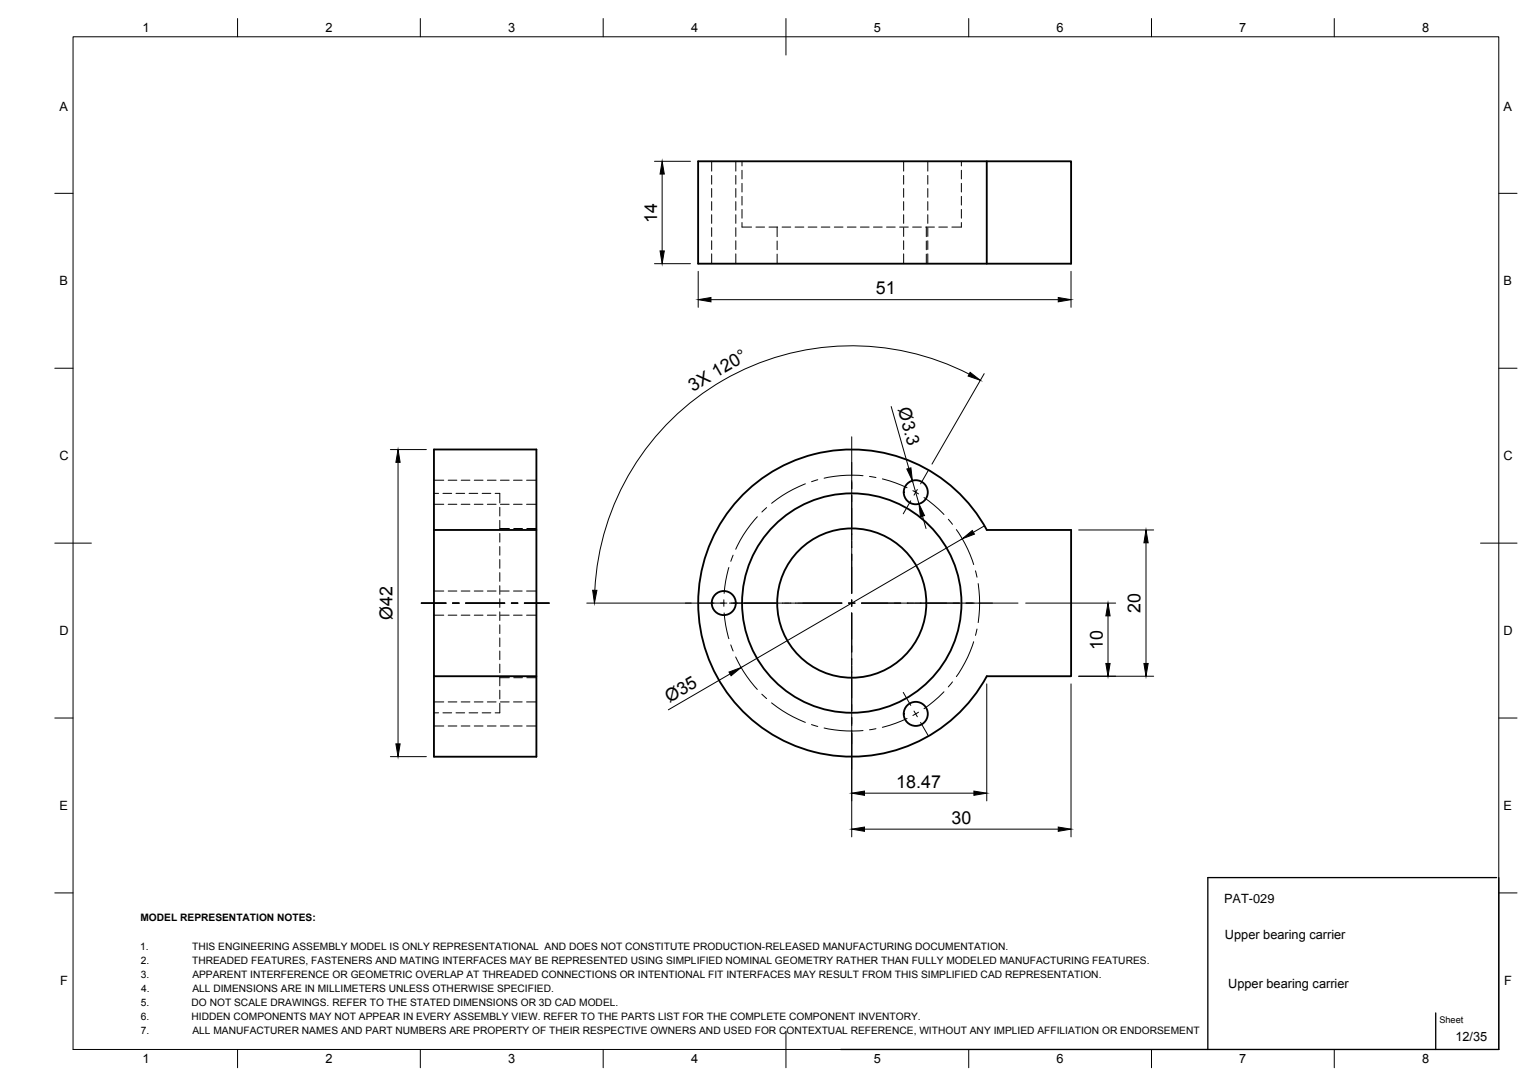
ISO-10303-21;
HEADER;
/* Generated by software containing ST-Developer
 * from STEP Tools, Inc. (www.steptools.com) 
 */

FILE_DESCRIPTION(
/* description */ ('Door-style hinge test fixture with detent'),
/* implementation_level */ '2;1');

FILE_NAME(
/* name */ 'Upper bearing carrier.step',
/* time_stamp */ '2026-10-28T03:24:57-07:00',
/* author */ (''),
/* organization */ (''),
/* preprocessor_version */ 'ST-DEVELOPER v20.2',
/* originating_system */ 'Autodesk Translation Framework v15.17.0.0',
/* authorisation */ '');

FILE_SCHEMA (('AUTOMOTIVE_DESIGN { 1 0 10303 214 3 1 1 }'));
ENDSEC;

DATA;
#10=MECHANICAL_DESIGN_GEOMETRIC_PRESENTATION_REPRESENTATION('',(#330),#9813);
#267=SHAPE_REPRESENTATION_RELATIONSHIP('SRR','None',#9944,#298);
#298=ADVANCED_BREP_SHAPE_REPRESENTATION('',(#370),#9787);
#330=STYLED_ITEM('',(#10183),#370);
#370=MANIFOLD_SOLID_BREP('Body1',#4761);
#440=FACE_BOUND('',#1067,.T.);
#441=FACE_BOUND('',#1070,.T.);
#442=FACE_BOUND('',#1071,.T.);
#443=FACE_BOUND('',#1072,.T.);
#444=FACE_BOUND('',#1073,.T.);
#445=FACE_BOUND('',#1079,.T.);
#446=FACE_BOUND('',#1080,.T.);
#447=FACE_BOUND('',#1081,.T.);
#448=FACE_BOUND('',#1082,.T.);
#547=PLANE('',#5291);
#548=PLANE('',#5295);
#549=PLANE('',#5297);
#550=PLANE('',#5298);
#551=PLANE('',#5299);
#552=PLANE('',#5302);
#736=FACE_OUTER_BOUND('',#1062,.T.);
#737=FACE_OUTER_BOUND('',#1063,.T.);
#738=FACE_OUTER_BOUND('',#1064,.T.);
#739=FACE_OUTER_BOUND('',#1065,.T.);
#740=FACE_OUTER_BOUND('',#1066,.T.);
#741=FACE_OUTER_BOUND('',#1068,.T.);
#742=FACE_OUTER_BOUND('',#1069,.T.);
#743=FACE_OUTER_BOUND('',#1074,.T.);
#744=FACE_OUTER_BOUND('',#1075,.T.);
#745=FACE_OUTER_BOUND('',#1076,.T.);
#746=FACE_OUTER_BOUND('',#1077,.T.);
#747=FACE_OUTER_BOUND('',#1078,.T.);
#1062=EDGE_LOOP('',(#3543,#3544,#3545,#3546));
#1063=EDGE_LOOP('',(#3547,#3548,#3549,#3550));
#1064=EDGE_LOOP('',(#3551,#3552,#3553,#3554));
#1065=EDGE_LOOP('',(#3555,#3556,#3557,#3558));
#1066=EDGE_LOOP('',(#3559));
#1067=EDGE_LOOP('',(#3560));
#1068=EDGE_LOOP('',(#3561,#3562,#3563,#3564));
#1069=EDGE_LOOP('',(#3565,#3566,#3567,#3568));
#1070=EDGE_LOOP('',(#3569));
#1071=EDGE_LOOP('',(#3570));
#1072=EDGE_LOOP('',(#3571));
#1073=EDGE_LOOP('',(#3572));
#1074=EDGE_LOOP('',(#3573,#3574,#3575,#3576));
#1075=EDGE_LOOP('',(#3577,#3578,#3579,#3580));
#1076=EDGE_LOOP('',(#3581,#3582,#3583,#3584));
#1077=EDGE_LOOP('',(#3585,#3586,#3587,#3588));
#1078=EDGE_LOOP('',(#3589,#3590,#3591,#3592));
#1079=EDGE_LOOP('',(#3593));
#1080=EDGE_LOOP('',(#3594));
#1081=EDGE_LOOP('',(#3595));
#1082=EDGE_LOOP('',(#3596));
#1444=LINE('',#7664,#1764);
#1445=LINE('',#7670,#1765);
#1446=LINE('',#7676,#1766);
#1447=LINE('',#7682,#1767);
#1448=LINE('',#7689,#1768);
#1449=LINE('',#7694,#1769);
#1450=LINE('',#7696,#1770);
#1451=LINE('',#7698,#1771);
#1452=LINE('',#7702,#1772);
#1453=LINE('',#7704,#1773);
#1454=LINE('',#7705,#1774);
#1455=LINE('',#7708,#1775);
#1456=LINE('',#7710,#1776);
#1457=LINE('',#7711,#1777);
#1458=LINE('',#7713,#1778);
#1764=VECTOR('',#6147,0.165);
#1765=VECTOR('',#6154,0.165);
#1766=VECTOR('',#6161,0.165);
#1767=VECTOR('',#6168,1.5);
#1768=VECTOR('',#6177,1.02);
#1769=VECTOR('',#6182,1.);
#1770=VECTOR('',#6183,1.);
#1771=VECTOR('',#6184,1.);
#1772=VECTOR('',#6189,1.);
#1773=VECTOR('',#6190,1.);
#1774=VECTOR('',#6191,1.);
#1775=VECTOR('',#6194,1.);
#1776=VECTOR('',#6195,1.);
#1777=VECTOR('',#6196,1.);
#1778=VECTOR('',#6199,1.);
#2032=CIRCLE('',#5280,0.165);
#2033=CIRCLE('',#5281,0.165);
#2034=CIRCLE('',#5283,0.165);
#2035=CIRCLE('',#5284,0.165);
#2036=CIRCLE('',#5286,0.165);
#2037=CIRCLE('',#5287,0.165);
#2038=CIRCLE('',#5289,1.5);
#2039=CIRCLE('',#5290,1.5);
#2040=CIRCLE('',#5292,1.02);
#2041=CIRCLE('',#5294,1.02);
#2042=CIRCLE('',#5296,2.1);
#2043=CIRCLE('',#5301,2.1);
#2333=VERTEX_POINT('',#7661);
#2334=VERTEX_POINT('',#7663);
#2335=VERTEX_POINT('',#7667);
#2336=VERTEX_POINT('',#7669);
#2337=VERTEX_POINT('',#7673);
#2338=VERTEX_POINT('',#7675);
#2339=VERTEX_POINT('',#7679);
#2340=VERTEX_POINT('',#7681);
#2341=VERTEX_POINT('',#7685);
#2342=VERTEX_POINT('',#7688);
#2343=VERTEX_POINT('',#7692);
#2344=VERTEX_POINT('',#7693);
#2345=VERTEX_POINT('',#7695);
#2346=VERTEX_POINT('',#7697);
#2347=VERTEX_POINT('',#7701);
#2348=VERTEX_POINT('',#7703);
#2349=VERTEX_POINT('',#7707);
#2350=VERTEX_POINT('',#7709);
#2788=EDGE_CURVE('',#2333,#2333,#2032,.T.);
#2789=EDGE_CURVE('',#2333,#2334,#1444,.T.);
#2790=EDGE_CURVE('',#2334,#2334,#2033,.T.);
#2791=EDGE_CURVE('',#2335,#2335,#2034,.T.);
#2792=EDGE_CURVE('',#2335,#2336,#1445,.T.);
#2793=EDGE_CURVE('',#2336,#2336,#2035,.T.);
#2794=EDGE_CURVE('',#2337,#2337,#2036,.T.);
#2795=EDGE_CURVE('',#2337,#2338,#1446,.T.);
#2796=EDGE_CURVE('',#2338,#2338,#2037,.T.);
#2797=EDGE_CURVE('',#2339,#2339,#2038,.T.);
#2798=EDGE_CURVE('',#2339,#2340,#1447,.T.);
#2799=EDGE_CURVE('',#2340,#2340,#2039,.T.);
#2800=EDGE_CURVE('',#2341,#2341,#2040,.T.);
#2801=EDGE_CURVE('',#2341,#2342,#1448,.T.);
#2802=EDGE_CURVE('',#2342,#2342,#2041,.T.);
#2803=EDGE_CURVE('',#2343,#2344,#1449,.T.);
#2804=EDGE_CURVE('',#2344,#2345,#1450,.T.);
#2805=EDGE_CURVE('',#2345,#2346,#1451,.T.);
#2806=EDGE_CURVE('',#2346,#2343,#2042,.T.);
#2807=EDGE_CURVE('',#2347,#2343,#1452,.T.);
#2808=EDGE_CURVE('',#2347,#2348,#1453,.T.);
#2809=EDGE_CURVE('',#2348,#2344,#1454,.T.);
#2810=EDGE_CURVE('',#2346,#2349,#1455,.T.);
#2811=EDGE_CURVE('',#2350,#2345,#1456,.T.);
#2812=EDGE_CURVE('',#2350,#2349,#1457,.T.);
#2813=EDGE_CURVE('',#2348,#2350,#1458,.T.);
#2814=EDGE_CURVE('',#2349,#2347,#2043,.T.);
#3543=ORIENTED_EDGE('',*,*,#2788,.F.);
#3544=ORIENTED_EDGE('',*,*,#2789,.T.);
#3545=ORIENTED_EDGE('',*,*,#2790,.F.);
#3546=ORIENTED_EDGE('',*,*,#2789,.F.);
#3547=ORIENTED_EDGE('',*,*,#2791,.F.);
#3548=ORIENTED_EDGE('',*,*,#2792,.T.);
#3549=ORIENTED_EDGE('',*,*,#2793,.F.);
#3550=ORIENTED_EDGE('',*,*,#2792,.F.);
#3551=ORIENTED_EDGE('',*,*,#2794,.F.);
#3552=ORIENTED_EDGE('',*,*,#2795,.T.);
#3553=ORIENTED_EDGE('',*,*,#2796,.F.);
#3554=ORIENTED_EDGE('',*,*,#2795,.F.);
#3555=ORIENTED_EDGE('',*,*,#2797,.F.);
#3556=ORIENTED_EDGE('',*,*,#2798,.T.);
#3557=ORIENTED_EDGE('',*,*,#2799,.T.);
#3558=ORIENTED_EDGE('',*,*,#2798,.F.);
#3559=ORIENTED_EDGE('',*,*,#2799,.F.);
#3560=ORIENTED_EDGE('',*,*,#2800,.F.);
#3561=ORIENTED_EDGE('',*,*,#2800,.T.);
#3562=ORIENTED_EDGE('',*,*,#2801,.T.);
#3563=ORIENTED_EDGE('',*,*,#2802,.F.);
#3564=ORIENTED_EDGE('',*,*,#2801,.F.);
#3565=ORIENTED_EDGE('',*,*,#2803,.T.);
#3566=ORIENTED_EDGE('',*,*,#2804,.T.);
#3567=ORIENTED_EDGE('',*,*,#2805,.T.);
#3568=ORIENTED_EDGE('',*,*,#2806,.T.);
#3569=ORIENTED_EDGE('',*,*,#2790,.T.);
#3570=ORIENTED_EDGE('',*,*,#2793,.T.);
#3571=ORIENTED_EDGE('',*,*,#2796,.T.);
#3572=ORIENTED_EDGE('',*,*,#2802,.T.);
#3573=ORIENTED_EDGE('',*,*,#2807,.F.);
#3574=ORIENTED_EDGE('',*,*,#2808,.T.);
#3575=ORIENTED_EDGE('',*,*,#2809,.T.);
#3576=ORIENTED_EDGE('',*,*,#2803,.F.);
#3577=ORIENTED_EDGE('',*,*,#2810,.F.);
#3578=ORIENTED_EDGE('',*,*,#2805,.F.);
#3579=ORIENTED_EDGE('',*,*,#2811,.F.);
#3580=ORIENTED_EDGE('',*,*,#2812,.T.);
#3581=ORIENTED_EDGE('',*,*,#2813,.T.);
#3582=ORIENTED_EDGE('',*,*,#2811,.T.);
#3583=ORIENTED_EDGE('',*,*,#2804,.F.);
#3584=ORIENTED_EDGE('',*,*,#2809,.F.);
#3585=ORIENTED_EDGE('',*,*,#2807,.T.);
#3586=ORIENTED_EDGE('',*,*,#2806,.F.);
#3587=ORIENTED_EDGE('',*,*,#2810,.T.);
#3588=ORIENTED_EDGE('',*,*,#2814,.T.);
#3589=ORIENTED_EDGE('',*,*,#2814,.F.);
#3590=ORIENTED_EDGE('',*,*,#2812,.F.);
#3591=ORIENTED_EDGE('',*,*,#2813,.F.);
#3592=ORIENTED_EDGE('',*,*,#2808,.F.);
#3593=ORIENTED_EDGE('',*,*,#2788,.T.);
#3594=ORIENTED_EDGE('',*,*,#2791,.T.);
#3595=ORIENTED_EDGE('',*,*,#2794,.T.);
#3596=ORIENTED_EDGE('',*,*,#2797,.T.);
#4407=CYLINDRICAL_SURFACE('',#5279,0.165);
#4408=CYLINDRICAL_SURFACE('',#5282,0.165);
#4409=CYLINDRICAL_SURFACE('',#5285,0.165);
#4410=CYLINDRICAL_SURFACE('',#5288,1.5);
#4411=CYLINDRICAL_SURFACE('',#5293,1.02);
#4412=CYLINDRICAL_SURFACE('',#5300,2.1);
#4541=ADVANCED_FACE('',(#736),#4407,.F.);
#4542=ADVANCED_FACE('',(#737),#4408,.F.);
#4543=ADVANCED_FACE('',(#738),#4409,.F.);
#4544=ADVANCED_FACE('',(#739),#4410,.F.);
#4545=ADVANCED_FACE('',(#740,#440),#547,.F.);
#4546=ADVANCED_FACE('',(#741),#4411,.F.);
#4547=ADVANCED_FACE('',(#742,#441,#442,#443,#444),#548,.T.);
#4548=ADVANCED_FACE('',(#743),#549,.T.);
#4549=ADVANCED_FACE('',(#744),#550,.T.);
#4550=ADVANCED_FACE('',(#745),#551,.T.);
#4551=ADVANCED_FACE('',(#746),#4412,.T.);
#4552=ADVANCED_FACE('',(#747,#445,#446,#447,#448),#552,.F.);
#4761=CLOSED_SHELL('',(#4541,#4542,#4543,#4544,#4545,#4546,#4547,#4548,
#4549,#4550,#4551,#4552));
#5278=AXIS2_PLACEMENT_3D('',#7659,#6141,#6142);
#5279=AXIS2_PLACEMENT_3D('',#7660,#6143,#6144);
#5280=AXIS2_PLACEMENT_3D('',#7662,#6145,#6146);
#5281=AXIS2_PLACEMENT_3D('',#7665,#6148,#6149);
#5282=AXIS2_PLACEMENT_3D('',#7666,#6150,#6151);
#5283=AXIS2_PLACEMENT_3D('',#7668,#6152,#6153);
#5284=AXIS2_PLACEMENT_3D('',#7671,#6155,#6156);
#5285=AXIS2_PLACEMENT_3D('',#7672,#6157,#6158);
#5286=AXIS2_PLACEMENT_3D('',#7674,#6159,#6160);
#5287=AXIS2_PLACEMENT_3D('',#7677,#6162,#6163);
#5288=AXIS2_PLACEMENT_3D('',#7678,#6164,#6165);
#5289=AXIS2_PLACEMENT_3D('',#7680,#6166,#6167);
#5290=AXIS2_PLACEMENT_3D('',#7683,#6169,#6170);
#5291=AXIS2_PLACEMENT_3D('',#7684,#6171,#6172);
#5292=AXIS2_PLACEMENT_3D('',#7686,#6173,#6174);
#5293=AXIS2_PLACEMENT_3D('',#7687,#6175,#6176);
#5294=AXIS2_PLACEMENT_3D('',#7690,#6178,#6179);
#5295=AXIS2_PLACEMENT_3D('',#7691,#6180,#6181);
#5296=AXIS2_PLACEMENT_3D('',#7699,#6185,#6186);
#5297=AXIS2_PLACEMENT_3D('',#7700,#6187,#6188);
#5298=AXIS2_PLACEMENT_3D('',#7706,#6192,#6193);
#5299=AXIS2_PLACEMENT_3D('',#7712,#6197,#6198);
#5300=AXIS2_PLACEMENT_3D('',#7714,#6200,#6201);
#5301=AXIS2_PLACEMENT_3D('',#7715,#6202,#6203);
#5302=AXIS2_PLACEMENT_3D('',#7716,#6204,#6205);
#6141=DIRECTION('axis',(0.,0.,1.));
#6142=DIRECTION('refdir',(1.,0.,0.));
#6143=DIRECTION('center_axis',(0.,0.,1.));
#6144=DIRECTION('ref_axis',(1.,0.,0.));
#6145=DIRECTION('center_axis',(0.,0.,1.));
#6146=DIRECTION('ref_axis',(1.,0.,0.));
#6147=DIRECTION('',(0.,0.,1.));
#6148=DIRECTION('center_axis',(0.,0.,-1.));
#6149=DIRECTION('ref_axis',(1.,0.,0.));
#6150=DIRECTION('center_axis',(0.,0.,1.));
#6151=DIRECTION('ref_axis',(1.,0.,0.));
#6152=DIRECTION('center_axis',(0.,0.,1.));
#6153=DIRECTION('ref_axis',(1.,0.,0.));
#6154=DIRECTION('',(0.,0.,1.));
#6155=DIRECTION('center_axis',(0.,0.,-1.));
#6156=DIRECTION('ref_axis',(1.,0.,0.));
#6157=DIRECTION('center_axis',(0.,0.,1.));
#6158=DIRECTION('ref_axis',(1.,0.,0.));
#6159=DIRECTION('center_axis',(0.,0.,1.));
#6160=DIRECTION('ref_axis',(1.,0.,0.));
#6161=DIRECTION('',(0.,0.,1.));
#6162=DIRECTION('center_axis',(0.,0.,-1.));
#6163=DIRECTION('ref_axis',(1.,0.,0.));
#6164=DIRECTION('center_axis',(0.,0.,1.));
#6165=DIRECTION('ref_axis',(1.,0.,0.));
#6166=DIRECTION('center_axis',(0.,0.,1.));
#6167=DIRECTION('ref_axis',(1.,0.,0.));
#6168=DIRECTION('',(0.,0.,1.));
#6169=DIRECTION('center_axis',(0.,0.,1.));
#6170=DIRECTION('ref_axis',(1.,0.,0.));
#6171=DIRECTION('center_axis',(0.,0.,1.));
#6172=DIRECTION('ref_axis',(1.,0.,0.));
#6173=DIRECTION('center_axis',(0.,0.,-1.));
#6174=DIRECTION('ref_axis',(1.,0.,0.));
#6175=DIRECTION('center_axis',(0.,0.,1.));
#6176=DIRECTION('ref_axis',(1.,0.,0.));
#6177=DIRECTION('',(0.,0.,1.));
#6178=DIRECTION('center_axis',(0.,0.,-1.));
#6179=DIRECTION('ref_axis',(1.,0.,0.));
#6180=DIRECTION('center_axis',(0.,0.,1.));
#6181=DIRECTION('ref_axis',(1.,0.,0.));
#6182=DIRECTION('',(-1.,0.,0.));
#6183=DIRECTION('',(0.,-1.,0.));
#6184=DIRECTION('',(1.,0.,0.));
#6185=DIRECTION('center_axis',(0.,0.,1.));
#6186=DIRECTION('ref_axis',(1.,0.,0.));
#6187=DIRECTION('center_axis',(0.,1.,0.));
#6188=DIRECTION('ref_axis',(-1.,0.,0.));
#6189=DIRECTION('',(0.,0.,1.));
#6190=DIRECTION('',(-1.,0.,0.));
#6191=DIRECTION('',(0.,0.,1.));
#6192=DIRECTION('center_axis',(0.,-1.,0.));
#6193=DIRECTION('ref_axis',(1.,0.,0.));
#6194=DIRECTION('',(0.,0.,-1.));
#6195=DIRECTION('',(0.,0.,1.));
#6196=DIRECTION('',(1.,0.,0.));
#6197=DIRECTION('center_axis',(-1.,0.,0.));
#6198=DIRECTION('ref_axis',(0.,-1.,0.));
#6199=DIRECTION('',(0.,-1.,0.));
#6200=DIRECTION('center_axis',(0.,0.,1.));
#6201=DIRECTION('ref_axis',(1.,0.,0.));
#6202=DIRECTION('center_axis',(0.,0.,1.));
#6203=DIRECTION('ref_axis',(1.,0.,0.));
#6204=DIRECTION('center_axis',(0.,0.,1.));
#6205=DIRECTION('ref_axis',(1.,0.,0.));
#7659=CARTESIAN_POINT('',(0.,0.,0.));
#7660=CARTESIAN_POINT('Origin',(1.75,0.,10.5));
#7661=CARTESIAN_POINT('',(1.585,-2.02066721859313E-17,10.6));
#7662=CARTESIAN_POINT('Origin',(1.75,0.,10.6));
#7663=CARTESIAN_POINT('',(1.585,2.02066721859313E-17,12.));
#7664=CARTESIAN_POINT('',(1.585,-2.02066721859313E-17,10.5));
#7665=CARTESIAN_POINT('Origin',(1.75,0.,12.));
#7666=CARTESIAN_POINT('Origin',(-0.875,1.51554445662277,10.5));
#7667=CARTESIAN_POINT('',(-1.04,1.51554445662277,10.6));
#7668=CARTESIAN_POINT('Origin',(-0.875,1.51554445662277,10.6));
#7669=CARTESIAN_POINT('',(-1.04,1.51554445662277,12.));
#7670=CARTESIAN_POINT('',(-1.04,1.51554445662277,10.5));
#7671=CARTESIAN_POINT('Origin',(-0.875,1.51554445662277,12.));
#7672=CARTESIAN_POINT('Origin',(-0.875000000000001,-1.51554445662277,10.5));
#7673=CARTESIAN_POINT('',(-1.04,-1.51554445662277,10.6));
#7674=CARTESIAN_POINT('Origin',(-0.875000000000001,-1.51554445662277,10.6));
#7675=CARTESIAN_POINT('',(-1.04,-1.51554445662277,12.));
#7676=CARTESIAN_POINT('',(-1.04,-1.51554445662277,10.5));
#7677=CARTESIAN_POINT('Origin',(-0.875000000000001,-1.51554445662277,12.));
#7678=CARTESIAN_POINT('Origin',(0.,0.,10.5));
#7679=CARTESIAN_POINT('',(-1.5,-1.83697019872103E-16,10.6));
#7680=CARTESIAN_POINT('Origin',(0.,0.,10.6));
#7681=CARTESIAN_POINT('',(-1.5,-1.83697019872103E-16,11.5));
#7682=CARTESIAN_POINT('',(-1.5,-1.83697019872103E-16,10.5));
#7683=CARTESIAN_POINT('Origin',(0.,0.,11.5));
#7684=CARTESIAN_POINT('Origin',(0.,0.,11.5));
#7685=CARTESIAN_POINT('',(-1.02,1.2491397351303E-16,11.5));
#7686=CARTESIAN_POINT('Origin',(0.,0.,11.5));
#7687=CARTESIAN_POINT('Origin',(0.,0.,10.5));
#7688=CARTESIAN_POINT('',(-1.02,1.2491397351303E-16,12.));
#7689=CARTESIAN_POINT('',(-1.02,-1.2491397351303E-16,10.5));
#7690=CARTESIAN_POINT('Origin',(0.,0.,12.));
#7691=CARTESIAN_POINT('Origin',(0.,0.,12.));
#7692=CARTESIAN_POINT('',(-1.84661853126194,1.,12.));
#7693=CARTESIAN_POINT('',(-3.,1.,12.));
#7694=CARTESIAN_POINT('',(0.,1.,12.));
#7695=CARTESIAN_POINT('',(-3.,-1.,12.));
#7696=CARTESIAN_POINT('',(-3.,1.,12.));
#7697=CARTESIAN_POINT('',(-1.84661853126194,-1.,12.));
#7698=CARTESIAN_POINT('',(-3.,-1.,12.));
#7699=CARTESIAN_POINT('Origin',(0.,0.,12.));
#7700=CARTESIAN_POINT('Origin',(0.,1.,10.6));
#7701=CARTESIAN_POINT('',(-1.84661853126194,1.,10.6));
#7702=CARTESIAN_POINT('',(-1.84661853126194,1.,10.6));
#7703=CARTESIAN_POINT('',(-3.,1.,10.6));
#7704=CARTESIAN_POINT('',(0.,1.,10.6));
#7705=CARTESIAN_POINT('',(-3.,1.,10.6));
#7706=CARTESIAN_POINT('Origin',(-3.,-1.,10.6));
#7707=CARTESIAN_POINT('',(-1.84661853126194,-1.,10.6));
#7708=CARTESIAN_POINT('',(-1.84661853126194,-1.,10.6));
#7709=CARTESIAN_POINT('',(-3.,-1.,10.6));
#7710=CARTESIAN_POINT('',(-3.,-1.,10.6));
#7711=CARTESIAN_POINT('',(-3.,-1.,10.6));
#7712=CARTESIAN_POINT('Origin',(-3.,1.,10.6));
#7713=CARTESIAN_POINT('',(-3.,1.,10.6));
#7714=CARTESIAN_POINT('Origin',(0.,0.,10.6));
#7715=CARTESIAN_POINT('Origin',(0.,0.,10.6));
#7716=CARTESIAN_POINT('Origin',(0.,0.,10.6));
#9751=UNCERTAINTY_MEASURE_WITH_UNIT(LENGTH_MEASURE(0.001),#9814,
'DISTANCE_ACCURACY_VALUE',
'Maximum model space distance between geometric entities at asserted c
onnectivities');
#9777=UNCERTAINTY_MEASURE_WITH_UNIT(LENGTH_MEASURE(0.001),#9814,
'DISTANCE_ACCURACY_VALUE',
'Maximum model space distance between geometric entities at asserted c
onnectivities');
#9787=(
GEOMETRIC_REPRESENTATION_CONTEXT(3)
GLOBAL_UNCERTAINTY_ASSIGNED_CONTEXT((#9751))
GLOBAL_UNIT_ASSIGNED_CONTEXT((#9814,#9816,#9817))
REPRESENTATION_CONTEXT('','3D')
);
#9813=(
GEOMETRIC_REPRESENTATION_CONTEXT(3)
GLOBAL_UNCERTAINTY_ASSIGNED_CONTEXT((#9777))
GLOBAL_UNIT_ASSIGNED_CONTEXT((#9814,#9816,#9817))
REPRESENTATION_CONTEXT('','3D')
);
#9814=(
LENGTH_UNIT()
NAMED_UNIT(*)
SI_UNIT(.CENTI.,.METRE.)
);
#9816=(
NAMED_UNIT(*)
PLANE_ANGLE_UNIT()
SI_UNIT($,.RADIAN.)
);
#9817=(
NAMED_UNIT(*)
SI_UNIT($,.STERADIAN.)
SOLID_ANGLE_UNIT()
);
#9827=SHAPE_DEFINITION_REPRESENTATION(#9862,#9944);
#9862=PRODUCT_DEFINITION_SHAPE('',$,#9980);
#9944=SHAPE_REPRESENTATION('',(#5278),#9787);
#9970=PRODUCT_DEFINITION_CONTEXT('part definition',#10077,'design');
#9980=PRODUCT_DEFINITION('Upper bearing carrier',
'Upper bearing carrier',#10015,#9970);
#10015=PRODUCT_DEFINITION_FORMATION('',$,#10088);
#10077=APPLICATION_CONTEXT(
'Core Data for Automotive Mechanical Design Process');
#10078=PRODUCT_CONTEXT('part definition',#10077,'mechanical');
#10088=PRODUCT('Upper bearing carrier','Upper bearing carrier',
'Upper bearing carrier',(#10078));
#10177=COLOUR_RGB('Grey',0.48,0.52,0.57);
#10178=FILL_AREA_STYLE_COLOUR('',#10177);
#10179=FILL_AREA_STYLE('',(#10178));
#10180=SURFACE_STYLE_FILL_AREA(#10179);
#10181=SURFACE_SIDE_STYLE('',(#10180));
#10182=SURFACE_STYLE_USAGE(.BOTH.,#10181);
#10183=PRESENTATION_STYLE_ASSIGNMENT((#10182));
ENDSEC;
END-ISO-10303-21;
